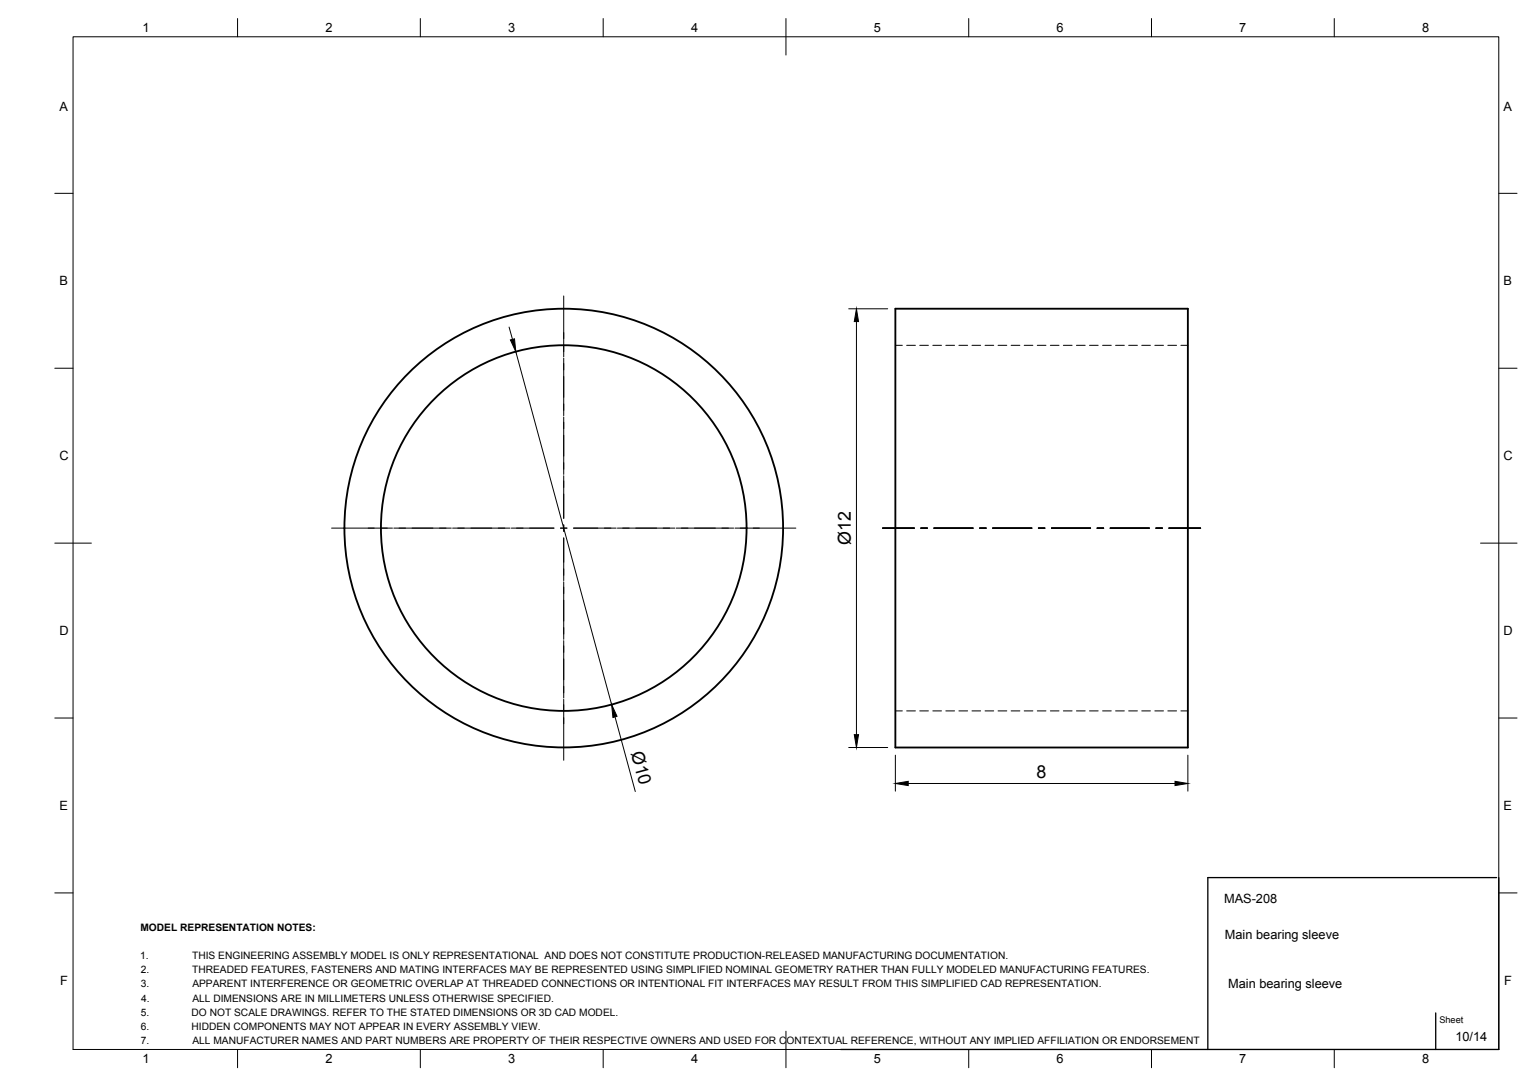
ISO-10303-21;
HEADER;
/* Generated by software containing ST-Developer
 * from STEP Tools, Inc. (www.steptools.com) 
 */

FILE_DESCRIPTION(
/* description */ ('Independent vertical20-tooth ratchet advance with repeated integral-c
ounterweight gravity pawls, swinging drive lever, bronze sleeves and f
ully retained axle stacks.18degpertooth. Native revolutes; geometric c
ycle checking rather than automatic contact/rolling dynamics. Gravity 
closing checked from actual pawl center of mass. Backplate/foot suppor
ts unit. Fits, torque, holding force, wear and life unassigned.'),
/* implementation_level */ '2;1');

FILE_NAME(
/* name */ 'Main bearing sleeve.step',
/* time_stamp */ '2026-11-09T06:25:53-08:00',
/* author */ (''),
/* organization */ (''),
/* preprocessor_version */ 'ST-DEVELOPER v20.2',
/* originating_system */ 'Autodesk Translation Framework v15.17.0.0',
/* authorisation */ '');

FILE_SCHEMA (('AUTOMOTIVE_DESIGN { 1 0 10303 214 3 1 1 }'));
ENDSEC;

DATA;
#10=MECHANICAL_DESIGN_GEOMETRIC_PRESENTATION_REPRESENTATION('',(#131),#4643);
#103=SHAPE_REPRESENTATION_RELATIONSHIP('SRR','None',#4708,#117);
#117=ADVANCED_BREP_SHAPE_REPRESENTATION('',(#145),#4637);
#131=STYLED_ITEM('',(#4785),#145);
#145=MANIFOLD_SOLID_BREP('Body1',#2667);
#182=FACE_BOUND('',#610,.T.);
#183=FACE_BOUND('',#612,.T.);
#290=PLANE('',#3017);
#291=PLANE('',#3018);
#427=FACE_OUTER_BOUND('',#607,.T.);
#428=FACE_OUTER_BOUND('',#608,.T.);
#429=FACE_OUTER_BOUND('',#609,.T.);
#430=FACE_OUTER_BOUND('',#611,.T.);
#607=EDGE_LOOP('',(#2389,#2390,#2391,#2392));
#608=EDGE_LOOP('',(#2393,#2394,#2395,#2396));
#609=EDGE_LOOP('',(#2397));
#610=EDGE_LOOP('',(#2398));
#611=EDGE_LOOP('',(#2399));
#612=EDGE_LOOP('',(#2400));
#887=LINE('',#4494,#1149);
#888=LINE('',#4500,#1150);
#1149=VECTOR('',#3701,5.);
#1150=VECTOR('',#3708,6.);
#1217=CIRCLE('',#3012,5.);
#1218=CIRCLE('',#3013,5.);
#1219=CIRCLE('',#3015,6.);
#1220=CIRCLE('',#3016,6.);
#1437=VERTEX_POINT('',#4491);
#1438=VERTEX_POINT('',#4493);
#1439=VERTEX_POINT('',#4497);
#1440=VERTEX_POINT('',#4499);
#1759=EDGE_CURVE('',#1437,#1437,#1217,.T.);
#1760=EDGE_CURVE('',#1437,#1438,#887,.T.);
#1761=EDGE_CURVE('',#1438,#1438,#1218,.T.);
#1762=EDGE_CURVE('',#1439,#1439,#1219,.T.);
#1763=EDGE_CURVE('',#1439,#1440,#888,.T.);
#1764=EDGE_CURVE('',#1440,#1440,#1220,.T.);
#2389=ORIENTED_EDGE('',*,*,#1759,.F.);
#2390=ORIENTED_EDGE('',*,*,#1760,.T.);
#2391=ORIENTED_EDGE('',*,*,#1761,.T.);
#2392=ORIENTED_EDGE('',*,*,#1760,.F.);
#2393=ORIENTED_EDGE('',*,*,#1762,.F.);
#2394=ORIENTED_EDGE('',*,*,#1763,.T.);
#2395=ORIENTED_EDGE('',*,*,#1764,.T.);
#2396=ORIENTED_EDGE('',*,*,#1763,.F.);
#2397=ORIENTED_EDGE('',*,*,#1762,.T.);
#2398=ORIENTED_EDGE('',*,*,#1759,.T.);
#2399=ORIENTED_EDGE('',*,*,#1764,.F.);
#2400=ORIENTED_EDGE('',*,*,#1761,.F.);
#2498=CYLINDRICAL_SURFACE('',#3011,5.);
#2499=CYLINDRICAL_SURFACE('',#3014,6.);
#2633=ADVANCED_FACE('',(#427),#2498,.F.);
#2634=ADVANCED_FACE('',(#428),#2499,.T.);
#2635=ADVANCED_FACE('',(#429,#182),#290,.T.);
#2636=ADVANCED_FACE('',(#430,#183),#291,.F.);
#2667=CLOSED_SHELL('',(#2633,#2634,#2635,#2636));
#3010=AXIS2_PLACEMENT_3D('',#4489,#3695,#3696);
#3011=AXIS2_PLACEMENT_3D('',#4490,#3697,#3698);
#3012=AXIS2_PLACEMENT_3D('',#4492,#3699,#3700);
#3013=AXIS2_PLACEMENT_3D('',#4495,#3702,#3703);
#3014=AXIS2_PLACEMENT_3D('',#4496,#3704,#3705);
#3015=AXIS2_PLACEMENT_3D('',#4498,#3706,#3707);
#3016=AXIS2_PLACEMENT_3D('',#4501,#3709,#3710);
#3017=AXIS2_PLACEMENT_3D('',#4502,#3711,#3712);
#3018=AXIS2_PLACEMENT_3D('',#4503,#3713,#3714);
#3695=DIRECTION('axis',(0.,0.,1.));
#3696=DIRECTION('refdir',(1.,0.,0.));
#3697=DIRECTION('center_axis',(0.,0.,1.));
#3698=DIRECTION('ref_axis',(1.,0.,0.));
#3699=DIRECTION('center_axis',(0.,0.,-1.));
#3700=DIRECTION('ref_axis',(1.,0.,0.));
#3701=DIRECTION('',(0.,0.,-1.));
#3702=DIRECTION('center_axis',(0.,0.,-1.));
#3703=DIRECTION('ref_axis',(1.,0.,0.));
#3704=DIRECTION('center_axis',(0.,0.,1.));
#3705=DIRECTION('ref_axis',(1.,0.,0.));
#3706=DIRECTION('center_axis',(0.,0.,1.));
#3707=DIRECTION('ref_axis',(1.,0.,0.));
#3708=DIRECTION('',(0.,0.,-1.));
#3709=DIRECTION('center_axis',(0.,0.,1.));
#3710=DIRECTION('ref_axis',(1.,0.,0.));
#3711=DIRECTION('center_axis',(0.,0.,1.));
#3712=DIRECTION('ref_axis',(1.,0.,0.));
#3713=DIRECTION('center_axis',(0.,0.,1.));
#3714=DIRECTION('ref_axis',(1.,0.,0.));
#4489=CARTESIAN_POINT('',(0.,0.,0.));
#4490=CARTESIAN_POINT('Origin',(0.,0.,0.));
#4491=CARTESIAN_POINT('',(-5.,-6.12323399573677E-16,8.));
#4492=CARTESIAN_POINT('Origin',(0.,0.,8.));
#4493=CARTESIAN_POINT('',(-5.,-6.12323399573677E-16,0.));
#4494=CARTESIAN_POINT('',(-5.,-6.12323399573677E-16,0.));
#4495=CARTESIAN_POINT('Origin',(0.,0.,0.));
#4496=CARTESIAN_POINT('Origin',(0.,0.,0.));
#4497=CARTESIAN_POINT('',(-6.,-7.34788079488412E-16,8.));
#4498=CARTESIAN_POINT('Origin',(0.,0.,8.));
#4499=CARTESIAN_POINT('',(-6.,-7.34788079488412E-16,0.));
#4500=CARTESIAN_POINT('',(-6.,-7.34788079488412E-16,0.));
#4501=CARTESIAN_POINT('Origin',(0.,0.,0.));
#4502=CARTESIAN_POINT('Origin',(0.,0.,8.));
#4503=CARTESIAN_POINT('Origin',(0.,0.,0.));
#4621=UNCERTAINTY_MEASURE_WITH_UNIT(LENGTH_MEASURE(0.01),#4644,
'DISTANCE_ACCURACY_VALUE',
'Maximum model space distance between geometric entities at asserted c
onnectivities');
#4627=UNCERTAINTY_MEASURE_WITH_UNIT(LENGTH_MEASURE(0.01),#4644,
'DISTANCE_ACCURACY_VALUE',
'Maximum model space distance between geometric entities at asserted c
onnectivities');
#4637=(
GEOMETRIC_REPRESENTATION_CONTEXT(3)
GLOBAL_UNCERTAINTY_ASSIGNED_CONTEXT((#4621))
GLOBAL_UNIT_ASSIGNED_CONTEXT((#4644,#4646,#4647))
REPRESENTATION_CONTEXT('','3D')
);
#4643=(
GEOMETRIC_REPRESENTATION_CONTEXT(3)
GLOBAL_UNCERTAINTY_ASSIGNED_CONTEXT((#4627))
GLOBAL_UNIT_ASSIGNED_CONTEXT((#4644,#4646,#4647))
REPRESENTATION_CONTEXT('','3D')
);
#4644=(
LENGTH_UNIT()
NAMED_UNIT(*)
SI_UNIT(.MILLI.,.METRE.)
);
#4646=(
NAMED_UNIT(*)
PLANE_ANGLE_UNIT()
SI_UNIT($,.RADIAN.)
);
#4647=(
NAMED_UNIT(*)
SI_UNIT($,.STERADIAN.)
SOLID_ANGLE_UNIT()
);
#4657=SHAPE_DEFINITION_REPRESENTATION(#4672,#4708);
#4672=PRODUCT_DEFINITION_SHAPE('',$,#4724);
#4708=SHAPE_REPRESENTATION('',(#3010),#4637);
#4714=PRODUCT_DEFINITION_CONTEXT('part definition',#4761,'design');
#4724=PRODUCT_DEFINITION('Main bearing sleeve','Main bearing sleeve',#4739,
#4714);
#4739=PRODUCT_DEFINITION_FORMATION('',$,#4772);
#4761=APPLICATION_CONTEXT(
'Core Data for Automotive Mechanical Design Process');
#4762=PRODUCT_CONTEXT('part definition',#4761,'mechanical');
#4772=PRODUCT('Main bearing sleeve','Main bearing sleeve',$,(#4762));
#4785=PRESENTATION_STYLE_ASSIGNMENT((#4794));
#4794=SURFACE_STYLE_USAGE(.BOTH.,#4803);
#4803=SURFACE_SIDE_STYLE('',(#4812));
#4812=SURFACE_STYLE_FILL_AREA(#4821);
#4821=FILL_AREA_STYLE('Bearing light gray',(#4830));
#4830=FILL_AREA_STYLE_COLOUR('Bearing light gray',#4839);
#4839=COLOUR_RGB('Bearing light gray',0.725490196078431,0.752941176470588,
0.792156862745098);
ENDSEC;
END-ISO-10303-21;
